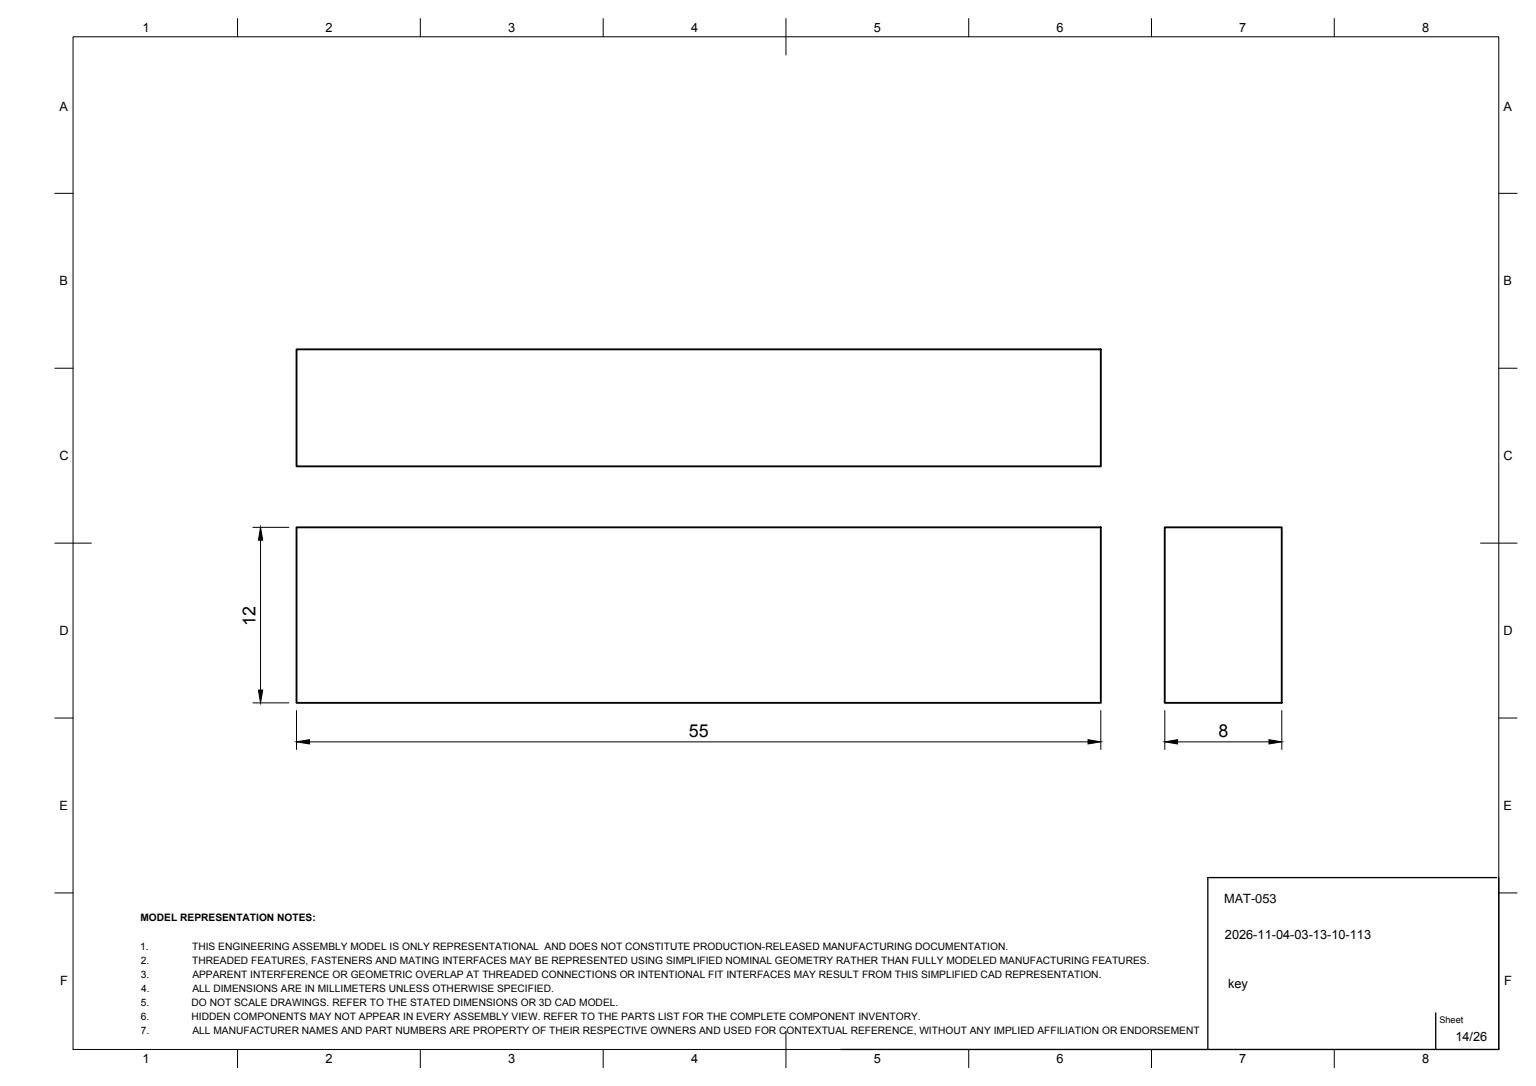
ISO-10303-21;
HEADER;
FILE_DESCRIPTION (('STEP AP214'),
    '1' );
FILE_NAME ('key.step',
    '2026-10-10T03:43:58',
    ( '' ),
    ( '' ),
    'SwSTEP 2.0',
    'SolidWorks 2026',
    '' );
FILE_SCHEMA (( 'AUTOMOTIVE_DESIGN' ));
ENDSEC;

DATA;
#429=( NAMED_UNIT ( * ) SI_UNIT ( $, .STERADIAN. ) SOLID_ANGLE_UNIT ( ) );
#674=ORIENTED_EDGE ( 'NONE', *, *, #10621, .T. ) ;
#812=ORIENTED_EDGE ( 'NONE', *, *, #10621, .F. ) ;
#867=FILL_AREA_STYLE ('',( #64184 ) ) ;
#916=DIRECTION ( 'NONE',  ( 1.261617073437677999E-16, 0.000000000000000000, 1.000000000000000000 ) ) ;
#2036=CARTESIAN_POINT ( 'NONE',  ( -5.066666666666671759, 0.000000000000000000, -11.86666666666666536 ) ) ;
#3000=DIRECTION ( 'NONE',  ( -1.261617073437677999E-16, 0.000000000000000000, -1.000000000000000000 ) ) ;
#4083=CARTESIAN_POINT ( 'NONE',  ( -5.066666666666671759, 0.000000000000000000, -11.86666666666666536 ) ) ;
#4386=CARTESIAN_POINT ( 'NONE',  ( -5.066666666666664653, 8.000000000000000000, 43.13333333333333286 ) ) ;
#4510=LINE ( 'NONE', #10469, #38529 ) ;
#5535=EDGE_CURVE ( 'NONE', #52890, #16495, #50210, .T. ) ;
#5609=ORIENTED_EDGE ( 'NONE', *, *, #42487, .F. ) ;
#5677=CARTESIAN_POINT ( 'NONE',  ( -5.066666666666671759, 0.000000000000000000, -11.86666666666666536 ) ) ;
#5782=( LENGTH_UNIT ( ) NAMED_UNIT ( * ) SI_UNIT ( .MILLI., .METRE. ) );
#6316=LINE ( 'NONE', #16174, #20001 ) ;
#6336=ORIENTED_EDGE ( 'NONE', *, *, #37384, .F. ) ;
#6541=CARTESIAN_POINT ( 'NONE',  ( -5.066666666666671759, 8.000000000000000000, -11.86666666666666536 ) ) ;
#6650=EDGE_LOOP ( 'NONE', ( #56529, #21988, #47611, #58341 ) ) ;
#6767=PLANE ( 'NONE',  #54681 ) ;
#7444=CARTESIAN_POINT ( 'NONE',  ( 6.933333333333335347, 8.000000000000000000, 43.13333333333333286 ) ) ;
#7507=CARTESIAN_POINT ( 'NONE',  ( -5.066666666666664653, 8.000000000000000000, 43.13333333333333286 ) ) ;
#8319=DIRECTION ( 'NONE',  ( 1.000000000000000000, 0.000000000000000000, 0.000000000000000000 ) ) ;
#9272=DIRECTION ( 'NONE',  ( -0.000000000000000000, -1.000000000000000000, -0.000000000000000000 ) ) ;
#9722=ORIENTED_EDGE ( 'NONE', *, *, #37384, .T. ) ;
#10017=ADVANCED_FACE ( 'NONE', ( #15627 ), #14253, .F. ) ;
#10128=DIRECTION ( 'NONE',  ( -1.261617073437677999E-16, -0.000000000000000000, -1.000000000000000000 ) ) ;
#10469=CARTESIAN_POINT ( 'NONE',  ( 6.933333333333328241, 0.000000000000000000, -11.86666666666666536 ) ) ;
#10592=LINE ( 'NONE', #64764, #41302 ) ;
#10621=EDGE_CURVE ( 'NONE', #16495, #58982, #10592, .T. ) ;
#11587=STYLED_ITEM ( 'NONE', ( #43412 ), #41290 ) ;
#11725=EDGE_CURVE ( 'NONE', #61254, #58982, #40475, .T. ) ;
#12936=DIRECTION ( 'NONE',  ( 1.261617073437677999E-16, 0.000000000000000000, 1.000000000000000000 ) ) ;
#13005=APPLICATION_CONTEXT ( 'automotive_design' ) ;
#13877=PRODUCT_DEFINITION ( 'UNKNOWN', '', #14187, #37353 ) ;
#13964=ORIENTED_EDGE ( 'NONE', *, *, #48199, .T. ) ;
#13976=CARTESIAN_POINT ( 'NONE',  ( -5.066666666666671759, 8.000000000000000000, -11.86666666666666536 ) ) ;
#14187=PRODUCT_DEFINITION_FORMATION_WITH_SPECIFIED_SOURCE ( 'ANY', '', #36615, .NOT_KNOWN. ) ;
#14253=PLANE ( 'NONE',  #16535 ) ;
#14967=MECHANICAL_DESIGN_GEOMETRIC_PRESENTATION_REPRESENTATION('',(#11587),#58787);
#15009=DIRECTION ( 'NONE',  ( -1.261617073437677999E-16, -0.000000000000000000, -1.000000000000000000 ) ) ;
#15210=CARTESIAN_POINT ( 'NONE',  ( -5.066666666666664653, 0.000000000000000000, 43.13333333333333286 ) ) ;
#15427=EDGE_LOOP ( 'NONE', ( #674, #62289, #24114, #9722 ) ) ;
#15627=FACE_OUTER_BOUND ( 'NONE', #15427, .T. ) ;
#16174=CARTESIAN_POINT ( 'NONE',  ( -5.066666666666664653, 8.000000000000000000, 43.13333333333333286 ) ) ;
#16495=VERTEX_POINT ( 'NONE', #15210 ) ;
#16535=AXIS2_PLACEMENT_3D ( 'NONE', #4386, #52562, #57505 ) ;
#16787=DIRECTION ( 'NONE',  ( -0.000000000000000000, -1.000000000000000000, -0.000000000000000000 ) ) ;
#16913=DIRECTION ( 'NONE',  ( 1.000000000000000000, 0.000000000000000000, 0.000000000000000000 ) ) ;
#17524=FACE_OUTER_BOUND ( 'NONE', #6650, .T. ) ;
#17715=PLANE ( 'NONE',  #51236 ) ;
#18562=DIRECTION ( 'NONE',  ( -1.000000000000000000, -0.000000000000000000, -0.000000000000000000 ) ) ;
#18706=PLANE ( 'NONE',  #50026 ) ;
#19554=ORIENTED_EDGE ( 'NONE', *, *, #25498, .T. ) ;
#19752=( GEOMETRIC_REPRESENTATION_CONTEXT ( 3 ) GLOBAL_UNCERTAINTY_ASSIGNED_CONTEXT ( ( #30370 ) ) GLOBAL_UNIT_ASSIGNED_CONTEXT ( ( #20501, #26481, #429 ) ) REPRESENTATION_CONTEXT ( 'NONE', 'WORKASPACE' ) );
#20001=VECTOR ( 'NONE', #58729, 1000.000000000000000 ) ;
#20007=DIRECTION ( 'NONE',  ( 0.000000000000000000, -0.000000000000000000, 1.000000000000000000 ) ) ;
#20501=( LENGTH_UNIT ( ) NAMED_UNIT ( * ) SI_UNIT ( .MILLI., .METRE. ) );
#20522=VERTEX_POINT ( 'NONE', #27022 ) ;
#20658=VECTOR ( 'NONE', #12936, 1000.000000000000000 ) ;
#20676=ADVANCED_BREP_SHAPE_REPRESENTATION ( '', ( #41290, #66832 ), #19752 ) ;
#20684=CARTESIAN_POINT ( 'NONE',  ( 0.000000000000000000, 8.000000000000000000, 0.000000000000000000 ) ) ;
#20946=PRODUCT_CONTEXT ( 'NONE', #13005, 'mechanical' ) ;
#20995=ADVANCED_FACE ( 'NONE', ( #17524 ), #29475, .F. ) ;
#21988=ORIENTED_EDGE ( 'NONE', *, *, #48720, .F. ) ;
#22595=CARTESIAN_POINT ( 'NONE',  ( 0.000000000000000000, 0.000000000000000000, 0.000000000000000000 ) ) ;
#23022=SURFACE_STYLE_FILL_AREA ( #867 ) ;
#23517=CARTESIAN_POINT ( 'NONE',  ( 6.933333333333328241, 8.000000000000000000, -11.86666666666666536 ) ) ;
#23649=DIRECTION ( 'NONE',  ( 0.000000000000000000, 1.000000000000000000, 0.000000000000000000 ) ) ;
#24114=ORIENTED_EDGE ( 'NONE', *, *, #48199, .F. ) ;
#24382=DIRECTION ( 'NONE',  ( 0.000000000000000000, 0.000000000000000000, 1.000000000000000000 ) ) ;
#24391=EDGE_LOOP ( 'NONE', ( #43584, #6336, #32989, #19554 ) ) ;
#24550=LINE ( 'NONE', #13976, #55542 ) ;
#24561=ADVANCED_FACE ( 'NONE', ( #37201 ), #18706, .T. ) ;
#25498=EDGE_CURVE ( 'NONE', #20522, #52890, #61274, .T. ) ;
#26481=( NAMED_UNIT ( * ) PLANE_ANGLE_UNIT ( ) SI_UNIT ( $, .RADIAN. ) );
#27022=CARTESIAN_POINT ( 'NONE',  ( -5.066666666666671759, 8.000000000000000000, -11.86666666666666536 ) ) ;
#27220=AXIS2_PLACEMENT_3D ( 'NONE', #23517, #45303, #60444 ) ;
#27608=VECTOR ( 'NONE', #916, 1000.000000000000000 ) ;
#28277=UNCERTAINTY_MEASURE_WITH_UNIT (LENGTH_MEASURE( 1.000000000000000082E-05 ), #5782, 'distance_accuracy_value', 'NONE');
#29475=PLANE ( 'NONE',  #27220 ) ;
#30215=ORIENTED_EDGE ( 'NONE', *, *, #5535, .F. ) ;
#30370=UNCERTAINTY_MEASURE_WITH_UNIT (LENGTH_MEASURE( 1.000000000000000082E-05 ), #20501, 'distance_accuracy_value', 'NONE');
#30970=APPLICATION_CONTEXT ( 'automotive_design' ) ;
#31422=CARTESIAN_POINT ( 'NONE',  ( -5.066666666666664653, 8.000000000000000000, 43.13333333333333286 ) ) ;
#32711=PRODUCT_DEFINITION_SHAPE ( 'NONE', 'NONE',  #13877 ) ;
#32989=ORIENTED_EDGE ( 'NONE', *, *, #44454, .F. ) ;
#33295=ADVANCED_FACE ( 'NONE', ( #39242 ), #44859, .F. ) ;
#33554=CARTESIAN_POINT ( 'NONE',  ( -5.066666666666671759, 8.000000000000000000, -11.86666666666666536 ) ) ;
#34564=CARTESIAN_POINT ( 'NONE',  ( -5.066666666666671759, 8.000000000000000000, -11.86666666666666536 ) ) ;
#34815=AXIS2_PLACEMENT_3D ( 'NONE', #45547, #55403, #3000 ) ;
#34932=FACE_OUTER_BOUND ( 'NONE', #40517, .T. ) ;
#34939=CARTESIAN_POINT ( 'NONE',  ( 6.933333333333335347, 0.000000000000000000, 43.13333333333333286 ) ) ;
#36391=CARTESIAN_POINT ( 'NONE',  ( 6.933333333333328241, 0.000000000000000000, -11.86666666666666536 ) ) ;
#36431=DIRECTION ( 'NONE',  ( -1.000000000000000000, -0.000000000000000000, -0.000000000000000000 ) ) ;
#36615=PRODUCT ( 'key', 'key', '', ( #20946 ) ) ;
#37050=EDGE_LOOP ( 'NONE', ( #30215, #39349, #69295, #812 ) ) ;
#37201=FACE_OUTER_BOUND ( 'NONE', #62943, .T. ) ;
#37353=PRODUCT_DEFINITION_CONTEXT ( 'detailed design', #30970, 'design' ) ;
#37361=SHAPE_REPRESENTATION_RELATIONSHIP ( 'NONE' , 'NONE' ,  #64925, #20676 ) ;
#37384=EDGE_CURVE ( 'NONE', #51166, #16495, #47576, .T. ) ;
#37445=( NAMED_UNIT ( * ) PLANE_ANGLE_UNIT ( ) SI_UNIT ( $, .RADIAN. ) );
#37802=SURFACE_STYLE_USAGE ( .BOTH. , #55014 ) ;
#38529=VECTOR ( 'NONE', #10128, 1000.000000000000000 ) ;
#38543=LINE ( 'NONE', #6541, #27608 ) ;
#38777=CARTESIAN_POINT ( 'NONE',  ( 6.933333333333328241, 8.000000000000000000, -11.86666666666666536 ) ) ;
#39242=FACE_OUTER_BOUND ( 'NONE', #24391, .T. ) ;
#39349=ORIENTED_EDGE ( 'NONE', *, *, #60161, .F. ) ;
#40402=ORIENTED_EDGE ( 'NONE', *, *, #25498, .F. ) ;
#40475=LINE ( 'NONE', #7444, #50342 ) ;
#40517=EDGE_LOOP ( 'NONE', ( #60442, #40402, #5609, #61827 ) ) ;
#40665=LINE ( 'NONE', #4083, #63585 ) ;
#40836=COLOUR_RGB ( '',0.7921568627450980005, 0.8196078431372548767, 0.9333333333333333481 ) ;
#41290=MANIFOLD_SOLID_BREP ( 'Boss-Extrude1', #48503 ) ;
#41302=VECTOR ( 'NONE', #16913, 1000.000000000000000 ) ;
#42054=SHAPE_DEFINITION_REPRESENTATION ( #32711, #64925 ) ;
#42487=EDGE_CURVE ( 'NONE', #60730, #20522, #24550, .T. ) ;
#42757=VERTEX_POINT ( 'NONE', #36391 ) ;
#43064=( NAMED_UNIT ( * ) SI_UNIT ( $, .STERADIAN. ) SOLID_ANGLE_UNIT ( ) );
#43412=PRESENTATION_STYLE_ASSIGNMENT (( #37802 ) ) ;
#43584=ORIENTED_EDGE ( 'NONE', *, *, #5535, .T. ) ;
#44306=ORIENTED_EDGE ( 'NONE', *, *, #42487, .T. ) ;
#44454=EDGE_CURVE ( 'NONE', #20522, #51166, #38543, .T. ) ;
#44558=DIRECTION ( 'NONE',  ( 0.000000000000000000, 0.000000000000000000, 1.000000000000000000 ) ) ;
#44755=DIRECTION ( 'NONE',  ( -0.000000000000000000, -1.000000000000000000, -0.000000000000000000 ) ) ;
#44859=PLANE ( 'NONE',  #34815 ) ;
#45121=ADVANCED_FACE ( 'NONE', ( #34932 ), #17715, .F. ) ;
#45303=DIRECTION ( 'NONE',  ( -1.000000000000000000, 0.000000000000000000, 1.261617073437677999E-16 ) ) ;
#45547=CARTESIAN_POINT ( 'NONE',  ( -5.066666666666671759, 8.000000000000000000, -11.86666666666666536 ) ) ;
#47576=LINE ( 'NONE', #31422, #65347 ) ;
#47611=ORIENTED_EDGE ( 'NONE', *, *, #57243, .F. ) ;
#48199=EDGE_CURVE ( 'NONE', #51166, #61254, #6316, .T. ) ;
#48503=CLOSED_SHELL ( 'NONE', ( #33295, #10017, #20995, #45121, #24561, #61684 ) ) ;
#48720=EDGE_CURVE ( 'NONE', #60730, #42757, #48778, .T. ) ;
#48778=LINE ( 'NONE', #64993, #67260 ) ;
#50026=AXIS2_PLACEMENT_3D ( 'NONE', #20684, #52008, #20007 ) ;
#50210=LINE ( 'NONE', #2036, #20658 ) ;
#50342=VECTOR ( 'NONE', #61595, 1000.000000000000000 ) ;
#50464=CARTESIAN_POINT ( 'NONE',  ( 6.933333333333335347, 8.000000000000000000, 43.13333333333333286 ) ) ;
#50530=CARTESIAN_POINT ( 'NONE',  ( 0.000000000000000000, 0.000000000000000000, 0.000000000000000000 ) ) ;
#51166=VERTEX_POINT ( 'NONE', #7507 ) ;
#51236=AXIS2_PLACEMENT_3D ( 'NONE', #33554, #24382, #56374 ) ;
#52008=DIRECTION ( 'NONE',  ( 0.000000000000000000, 1.000000000000000000, 0.000000000000000000 ) ) ;
#52562=DIRECTION ( 'NONE',  ( 0.000000000000000000, 0.000000000000000000, -1.000000000000000000 ) ) ;
#52890=VERTEX_POINT ( 'NONE', #5677 ) ;
#53292=ORIENTED_EDGE ( 'NONE', *, *, #44454, .T. ) ;
#54131=EDGE_CURVE ( 'NONE', #58982, #42757, #4510, .T. ) ;
#54681=AXIS2_PLACEMENT_3D ( 'NONE', #22595, #23649, #65520 ) ;
#54946=FACE_OUTER_BOUND ( 'NONE', #37050, .T. ) ;
#55014=SURFACE_SIDE_STYLE ('',( #23022 ) ) ;
#55349=ORIENTED_EDGE ( 'NONE', *, *, #57243, .T. ) ;
#55403=DIRECTION ( 'NONE',  ( 1.000000000000000000, 0.000000000000000000, -1.261617073437677999E-16 ) ) ;
#55542=VECTOR ( 'NONE', #18562, 1000.000000000000000 ) ;
#55703=VECTOR ( 'NONE', #44755, 1000.000000000000000 ) ;
#56374=DIRECTION ( 'NONE',  ( 1.000000000000000000, 0.000000000000000000, -0.000000000000000000 ) ) ;
#56529=ORIENTED_EDGE ( 'NONE', *, *, #54131, .T. ) ;
#57243=EDGE_CURVE ( 'NONE', #61254, #60730, #62861, .T. ) ;
#57505=DIRECTION ( 'NONE',  ( -1.000000000000000000, 0.000000000000000000, -0.000000000000000000 ) ) ;
#57585=CARTESIAN_POINT ( 'NONE',  ( 6.933333333333328241, 8.000000000000000000, -11.86666666666666536 ) ) ;
#58341=ORIENTED_EDGE ( 'NONE', *, *, #11725, .T. ) ;
#58729=DIRECTION ( 'NONE',  ( 1.000000000000000000, 0.000000000000000000, 0.000000000000000000 ) ) ;
#58787=( GEOMETRIC_REPRESENTATION_CONTEXT ( 3 ) GLOBAL_UNCERTAINTY_ASSIGNED_CONTEXT ( ( #28277 ) ) GLOBAL_UNIT_ASSIGNED_CONTEXT ( ( #5782, #37445, #43064 ) ) REPRESENTATION_CONTEXT ( 'NONE', 'WORKASPACE' ) );
#58982=VERTEX_POINT ( 'NONE', #34939 ) ;
#60161=EDGE_CURVE ( 'NONE', #42757, #52890, #40665, .T. ) ;
#60442=ORIENTED_EDGE ( 'NONE', *, *, #60161, .T. ) ;
#60444=DIRECTION ( 'NONE',  ( 1.261617073437677999E-16, 0.000000000000000000, 1.000000000000000000 ) ) ;
#60730=VERTEX_POINT ( 'NONE', #38777 ) ;
#61254=VERTEX_POINT ( 'NONE', #50464 ) ;
#61274=LINE ( 'NONE', #34564, #55703 ) ;
#61282=VECTOR ( 'NONE', #15009, 1000.000000000000000 ) ;
#61595=DIRECTION ( 'NONE',  ( -0.000000000000000000, -1.000000000000000000, -0.000000000000000000 ) ) ;
#61684=ADVANCED_FACE ( 'NONE', ( #54946 ), #6767, .F. ) ;
#61827=ORIENTED_EDGE ( 'NONE', *, *, #48720, .T. ) ;
#62289=ORIENTED_EDGE ( 'NONE', *, *, #11725, .F. ) ;
#62861=LINE ( 'NONE', #57585, #61282 ) ;
#62943=EDGE_LOOP ( 'NONE', ( #53292, #13964, #55349, #44306 ) ) ;
#63585=VECTOR ( 'NONE', #36431, 1000.000000000000000 ) ;
#64184=FILL_AREA_STYLE_COLOUR ( '', #40836 ) ;
#64764=CARTESIAN_POINT ( 'NONE',  ( -5.066666666666664653, 0.000000000000000000, 43.13333333333333286 ) ) ;
#64925=SHAPE_REPRESENTATION ( 'key', ( #66832 ), #19752 ) ;
#64993=CARTESIAN_POINT ( 'NONE',  ( 6.933333333333328241, 8.000000000000000000, -11.86666666666666536 ) ) ;
#65347=VECTOR ( 'NONE', #9272, 1000.000000000000000 ) ;
#65520=DIRECTION ( 'NONE',  ( 0.000000000000000000, -0.000000000000000000, 1.000000000000000000 ) ) ;
#66832=AXIS2_PLACEMENT_3D ( 'NONE', #50530, #44558, #8319 ) ;
#67260=VECTOR ( 'NONE', #16787, 1000.000000000000000 ) ;
#69295=ORIENTED_EDGE ( 'NONE', *, *, #54131, .F. ) ;
ENDSEC;
END-ISO-10303-21;
